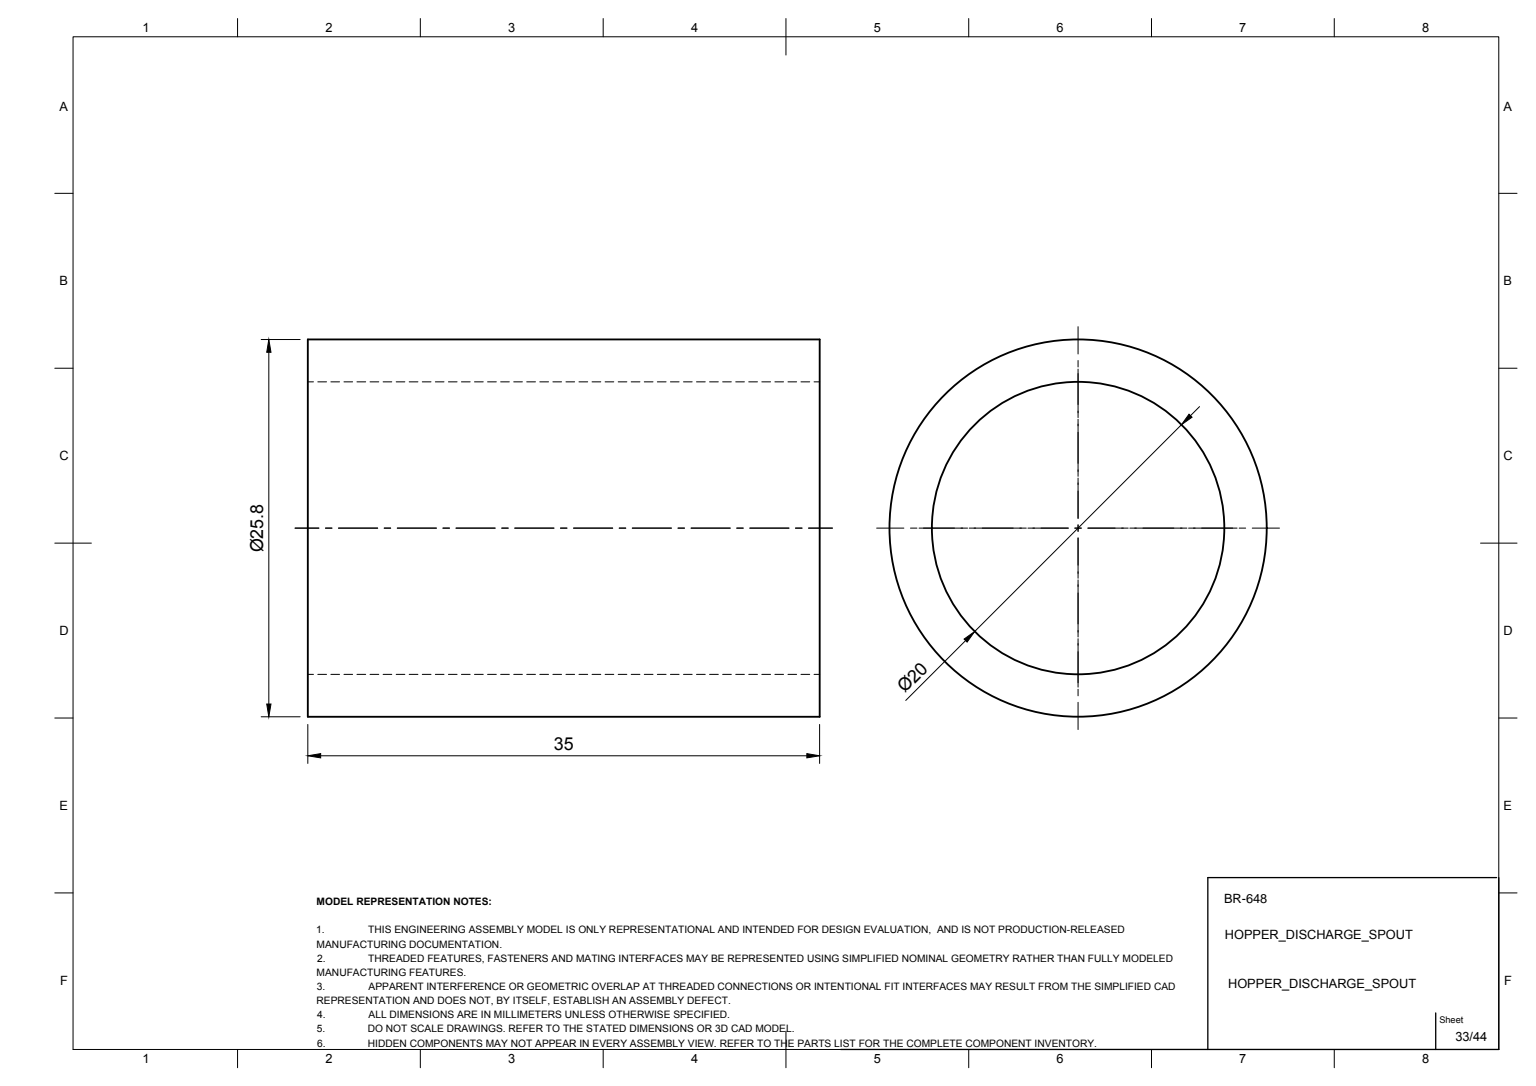
ISO-10303-21;
HEADER;
FILE_DESCRIPTION((''),'2;1');
FILE_NAME('HOPPER_DISCHARGE_SPOUT.step','2026-10-01T22:05:39-07:00',(''),(''),'','','');
FILE_SCHEMA (('AUTOMOTIVE_DESIGN { 1 0 10303 214 3 1 1 }'));
ENDSEC;
DATA;
#10=MECHANICAL_DESIGN_GEOMETRIC_PRESENTATION_REPRESENTATION('',(#631),#24628);
#547=SHAPE_REPRESENTATION_RELATIONSHIP('SRR','None',#24820,#589) ;
#589=ADVANCED_BREP_SHAPE_REPRESENTATION('',(#670),#24610) ;
#631=STYLED_ITEM('',(#25037),#670) ;
#670=MANIFOLD_SOLID_BREP('HOPPER_DISCHARGE_SPOUT',#13173) ;
#900=FACE_BOUND('',#4570,.T.) ;
#901=FACE_BOUND('',#4572,.T.) ;
#1666=LINE('',#23587,#2502) ;
#1667=LINE('',#23593,#2503) ;
#2502=VECTOR('',#18943,1.) ;
#2503=VECTOR('',#18950,1.29) ;
#2903=CYLINDRICAL_SURFACE('',#15094,1.) ;
#2904=CYLINDRICAL_SURFACE('',#15097,1.29) ;
#3586=FACE_OUTER_BOUND('',#4567,.T.) ;
#3587=FACE_OUTER_BOUND('',#4568,.T.) ;
#3588=FACE_OUTER_BOUND('',#4569,.T.) ;
#3589=FACE_OUTER_BOUND('',#4571,.T.) ;
#4567=EDGE_LOOP('',(#11411,#11412,#11413,#11414)) ;
#4568=EDGE_LOOP('',(#11415,#11416,#11417,#11418)) ;
#4569=EDGE_LOOP('',(#11419)) ;
#4570=EDGE_LOOP('',(#11420)) ;
#4571=EDGE_LOOP('',(#11421)) ;
#4572=EDGE_LOOP('',(#11422)) ;
#5439=CIRCLE('',#15095,1.) ;
#5440=CIRCLE('',#15096,1.) ;
#5441=CIRCLE('',#15098,1.29) ;
#5442=CIRCLE('',#15099,1.29) ;
#6541=VERTEX_POINT('',#23584) ;
#6542=VERTEX_POINT('',#23586) ;
#6543=VERTEX_POINT('',#23590) ;
#6544=VERTEX_POINT('',#23592) ;
#8195=EDGE_CURVE('',#6541,#6541,#5439,.T.) ;
#8196=EDGE_CURVE('',#6541,#6542,#1666,.T.) ;
#8197=EDGE_CURVE('',#6542,#6542,#5440,.T.) ;
#8198=EDGE_CURVE('',#6543,#6543,#5441,.T.) ;
#8199=EDGE_CURVE('',#6543,#6544,#1667,.T.) ;
#8200=EDGE_CURVE('',#6544,#6544,#5442,.T.) ;
#11411=ORIENTED_EDGE('',*,*,#8195,.F.) ;
#11412=ORIENTED_EDGE('',*,*,#8196,.T.) ;
#11413=ORIENTED_EDGE('',*,*,#8197,.F.) ;
#11414=ORIENTED_EDGE('',*,*,#8196,.F.) ;
#11415=ORIENTED_EDGE('',*,*,#8198,.F.) ;
#11416=ORIENTED_EDGE('',*,*,#8199,.T.) ;
#11417=ORIENTED_EDGE('',*,*,#8200,.F.) ;
#11418=ORIENTED_EDGE('',*,*,#8199,.F.) ;
#11419=ORIENTED_EDGE('',*,*,#8200,.T.) ;
#11420=ORIENTED_EDGE('',*,*,#8195,.T.) ;
#11421=ORIENTED_EDGE('',*,*,#8198,.T.) ;
#11422=ORIENTED_EDGE('',*,*,#8197,.T.) ;
#12268=PLANE('',#15100) ;
#12269=PLANE('',#15101) ;
#12981=ADVANCED_FACE('',(#3586),#2903,.F.) ;
#12982=ADVANCED_FACE('',(#3587),#2904,.T.) ;
#12983=ADVANCED_FACE('',(#3588,#900),#12268,.T.) ;
#12984=ADVANCED_FACE('',(#3589,#901),#12269,.T.) ;
#13173=CLOSED_SHELL('',(#12981,#12982,#12983,#12984)) ;
#15093=AXIS2_PLACEMENT_3D('',#23582,#18937,#18938) ;
#15094=AXIS2_PLACEMENT_3D('',#23583,#18939,#18940) ;
#15095=AXIS2_PLACEMENT_3D('',#23585,#18941,#18942) ;
#15096=AXIS2_PLACEMENT_3D('',#23588,#18944,#18945) ;
#15097=AXIS2_PLACEMENT_3D('',#23589,#18946,#18947) ;
#15098=AXIS2_PLACEMENT_3D('',#23591,#18948,#18949) ;
#15099=AXIS2_PLACEMENT_3D('',#23594,#18951,#18952) ;
#15100=AXIS2_PLACEMENT_3D('',#23595,#18953,#18954) ;
#15101=AXIS2_PLACEMENT_3D('',#23596,#18955,#18956) ;
#18937=DIRECTION('axis',(0.,0.,1.)) ;
#18938=DIRECTION('refdir',(1.,0.,0.)) ;
#18939=DIRECTION('center_axis',(0.,0.,1.)) ;
#18940=DIRECTION('ref_axis',(1.,0.,0.)) ;
#18941=DIRECTION('center_axis',(0.,0.,1.)) ;
#18942=DIRECTION('ref_axis',(1.,0.,0.)) ;
#18943=DIRECTION('',(0.,0.,1.)) ;
#18944=DIRECTION('center_axis',(0.,0.,-1.)) ;
#18945=DIRECTION('ref_axis',(1.,0.,0.)) ;
#18946=DIRECTION('center_axis',(0.,0.,1.)) ;
#18947=DIRECTION('ref_axis',(1.,0.,0.)) ;
#18948=DIRECTION('center_axis',(0.,0.,1.)) ;
#18949=DIRECTION('ref_axis',(1.,0.,0.)) ;
#18950=DIRECTION('',(0.,0.,-1.)) ;
#18951=DIRECTION('center_axis',(0.,0.,-1.)) ;
#18952=DIRECTION('ref_axis',(1.,0.,0.)) ;
#18953=DIRECTION('center_axis',(0.,0.,-1.)) ;
#18954=DIRECTION('ref_axis',(-1.,0.,0.)) ;
#18955=DIRECTION('center_axis',(0.,0.,1.)) ;
#18956=DIRECTION('ref_axis',(1.,0.,0.)) ;
#23582=CARTESIAN_POINT('',(0.,0.,0.)) ;
#23583=CARTESIAN_POINT('Origin',(-23.,-1.8,-5.75)) ;
#23584=CARTESIAN_POINT('',(-24.,-1.8,-7.5)) ;
#23585=CARTESIAN_POINT('Origin',(-23.,-1.8,-7.5)) ;
#23586=CARTESIAN_POINT('',(-24.,-1.8,-4.)) ;
#23587=CARTESIAN_POINT('',(-24.,-1.8,-5.75)) ;
#23588=CARTESIAN_POINT('Origin',(-23.,-1.8,-4.)) ;
#23589=CARTESIAN_POINT('Origin',(-23.,-1.8,-5.75)) ;
#23590=CARTESIAN_POINT('',(-24.29,-1.8,-4.)) ;
#23591=CARTESIAN_POINT('Origin',(-23.,-1.8,-4.)) ;
#23592=CARTESIAN_POINT('',(-24.29,-1.8,-7.5)) ;
#23593=CARTESIAN_POINT('',(-24.29,-1.8,-5.75)) ;
#23594=CARTESIAN_POINT('Origin',(-23.,-1.8,-7.5)) ;
#23595=CARTESIAN_POINT('Origin',(-23.,-1.8,-7.5)) ;
#23596=CARTESIAN_POINT('Origin',(-23.,-1.8,-4.)) ;
#24562=UNCERTAINTY_MEASURE_WITH_UNIT(LENGTH_MEASURE(0.001),#24629,
'DISTANCE_ACCURACY_VALUE',
'Maximum model space distance between geometric entities at asserted c
onnectivities') ;
#24580=UNCERTAINTY_MEASURE_WITH_UNIT(LENGTH_MEASURE(0.001),#24629,
'DISTANCE_ACCURACY_VALUE',
'Maximum model space distance between geometric entities at asserted c
onnectivities') ;
#24610=(
GEOMETRIC_REPRESENTATION_CONTEXT(3)
GLOBAL_UNCERTAINTY_ASSIGNED_CONTEXT((#24562))
GLOBAL_UNIT_ASSIGNED_CONTEXT((#24629,#24631,#24632))
REPRESENTATION_CONTEXT('','3D')
) ;
#24628=(
GEOMETRIC_REPRESENTATION_CONTEXT(3)
GLOBAL_UNCERTAINTY_ASSIGNED_CONTEXT((#24580))
GLOBAL_UNIT_ASSIGNED_CONTEXT((#24629,#24631,#24632))
REPRESENTATION_CONTEXT('','3D')
) ;
#24629=(
LENGTH_UNIT()
NAMED_UNIT(*)
SI_UNIT(.CENTI.,.METRE.)
) ;
#24631=(
NAMED_UNIT(*)
PLANE_ANGLE_UNIT()
SI_UNIT($,.RADIAN.)
) ;
#24632=(
NAMED_UNIT(*)
SI_UNIT($,.STERADIAN.)
SOLID_ANGLE_UNIT()
) ;
#24662=SHAPE_DEFINITION_REPRESENTATION(#24731,#24820) ;
#24731=PRODUCT_DEFINITION_SHAPE('',$,#24868) ;
#24820=SHAPE_REPRESENTATION('',(#15093),#24610) ;
#24838=PRODUCT_DEFINITION_CONTEXT('part definition',#24981,'design') ;
#24868=PRODUCT_DEFINITION('HOPPER_DISCHARGE_SPOUT',
'HOPPER_DISCHARGE_SPOUT',#24915,#24838) ;
#24915=PRODUCT_DEFINITION_FORMATION('',$,#25012) ;
#24981=APPLICATION_CONTEXT(
'Core Data for Automotive Mechanical Design Process') ;
#24982=PRODUCT_CONTEXT('part definition',#24981,'mechanical') ;
#25012=PRODUCT('HOPPER_DISCHARGE_SPOUT','HOPPER_DISCHARGE_SPOUT',$,(#24982)) ;
#25037=PRESENTATION_STYLE_ASSIGNMENT((#25047)) ;
#25047=SURFACE_STYLE_USAGE(.BOTH.,#25057) ;
#25057=SURFACE_SIDE_STYLE('',(#25067)) ;
#25067=SURFACE_STYLE_FILL_AREA(#25077) ;
#25077=FILL_AREA_STYLE('Steel - Galvanized (Small)',(#25087)) ;
#25087=FILL_AREA_STYLE_COLOUR('Steel - Galvanized (Small)',#25097) ;
#25097=COLOUR_RGB('Steel - Galvanized (Small)', 0.31764706, 0.68627451, 0.89019608) ;
ENDSEC;
END-ISO-10303-21;
